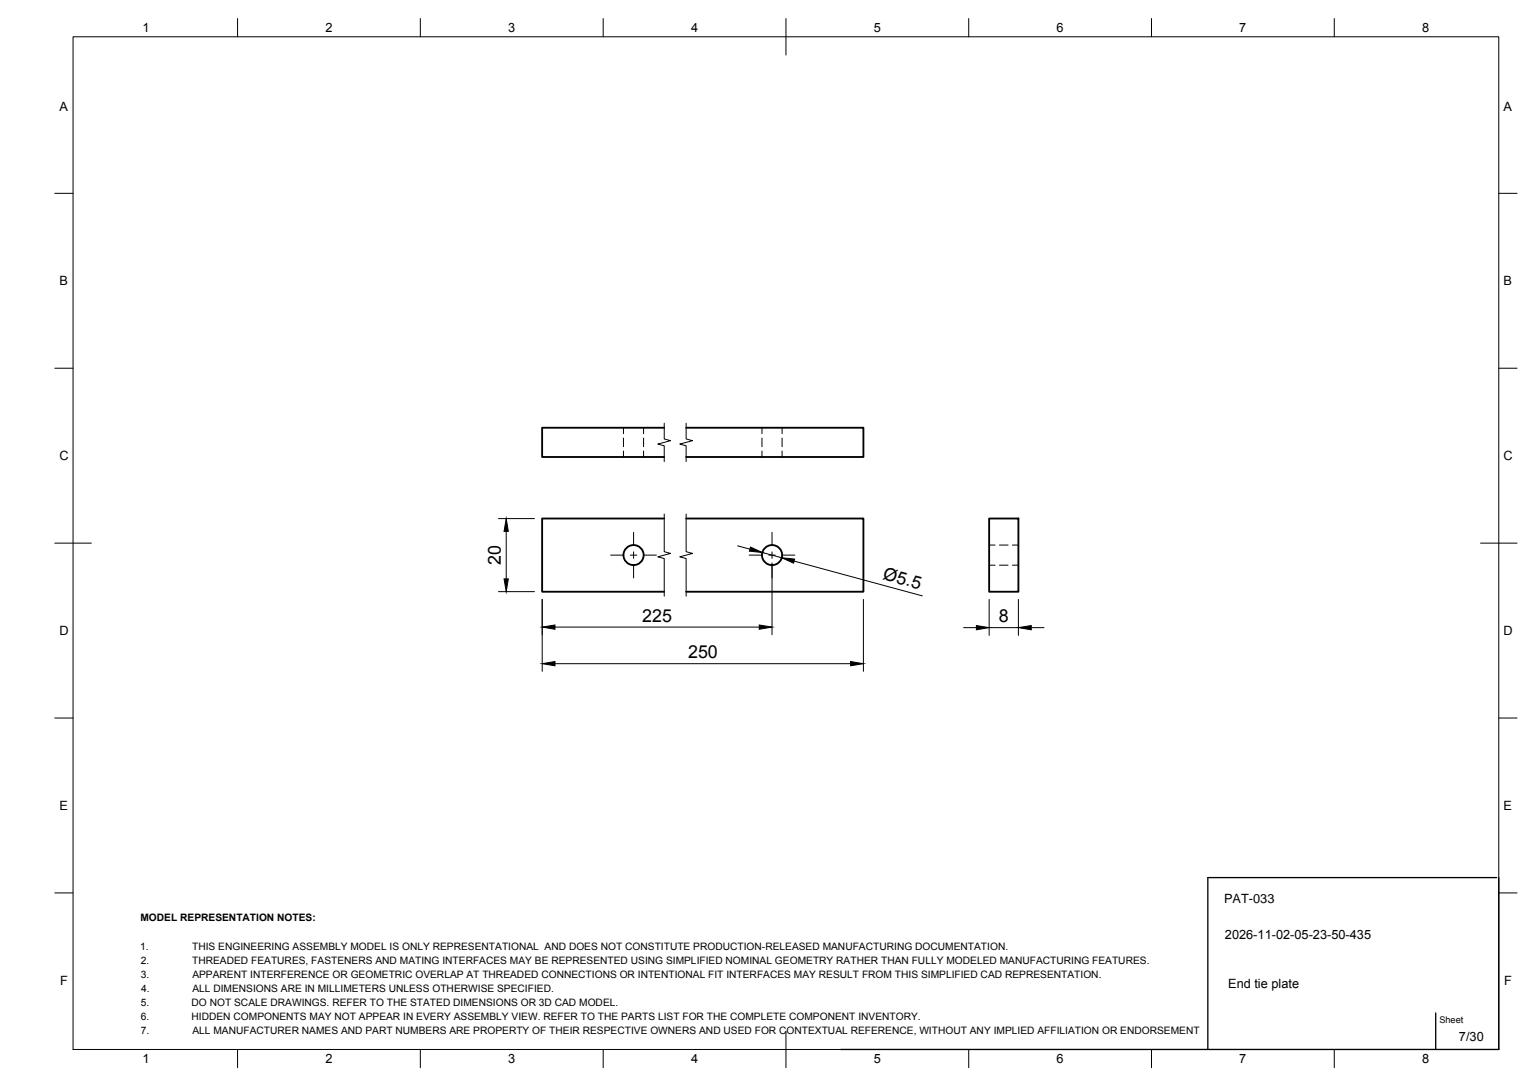
ISO-10303-21;
HEADER;
/* Generated by software containing ST-Developer
 * from STEP Tools, Inc. (www.steptools.com) 
 */

FILE_DESCRIPTION(
/* description */ ('Dual-rail gantry carriage'),
/* implementation_level */ '2;1');

FILE_NAME(
/* name */ 'End tie plate.step',
/* time_stamp */ '2026-10-27T10:49:15-07:00',
/* author */ (''),
/* organization */ (''),
/* preprocessor_version */ 'ST-DEVELOPER v20.2',
/* originating_system */ 'Autodesk Translation Framework v15.17.0.0',
/* authorisation */ '');

FILE_SCHEMA (('AUTOMOTIVE_DESIGN { 1 0 10303 214 3 1 1 }'));
ENDSEC;

DATA;
#10=MECHANICAL_DESIGN_GEOMETRIC_PRESENTATION_REPRESENTATION('',(#587),#12804);
#525=SHAPE_REPRESENTATION_RELATIONSHIP('SRR','None',#13003,#556);
#556=ADVANCED_BREP_SHAPE_REPRESENTATION('',(#618),#12773);
#587=STYLED_ITEM('',(#13233),#618);
#618=MANIFOLD_SOLID_BREP('Body1',#7365);
#666=FACE_BOUND('',#1492,.T.);
#667=FACE_BOUND('',#1493,.T.);
#668=FACE_BOUND('',#1495,.T.);
#669=FACE_BOUND('',#1496,.T.);
#776=PLANE('',#7800);
#777=PLANE('',#7801);
#778=PLANE('',#7802);
#779=PLANE('',#7803);
#780=PLANE('',#7804);
#781=PLANE('',#7805);
#1072=FACE_OUTER_BOUND('',#1485,.T.);
#1073=FACE_OUTER_BOUND('',#1486,.T.);
#1074=FACE_OUTER_BOUND('',#1487,.T.);
#1075=FACE_OUTER_BOUND('',#1488,.T.);
#1076=FACE_OUTER_BOUND('',#1489,.T.);
#1077=FACE_OUTER_BOUND('',#1490,.T.);
#1078=FACE_OUTER_BOUND('',#1491,.T.);
#1079=FACE_OUTER_BOUND('',#1494,.T.);
#1485=EDGE_LOOP('',(#5187,#5188,#5189,#5190));
#1486=EDGE_LOOP('',(#5191,#5192,#5193,#5194));
#1487=EDGE_LOOP('',(#5195,#5196,#5197,#5198));
#1488=EDGE_LOOP('',(#5199,#5200,#5201,#5202));
#1489=EDGE_LOOP('',(#5203,#5204,#5205,#5206));
#1490=EDGE_LOOP('',(#5207,#5208,#5209,#5210));
#1491=EDGE_LOOP('',(#5211,#5212,#5213,#5214));
#1492=EDGE_LOOP('',(#5215));
#1493=EDGE_LOOP('',(#5216));
#1494=EDGE_LOOP('',(#5217,#5218,#5219,#5220));
#1495=EDGE_LOOP('',(#5221));
#1496=EDGE_LOOP('',(#5222));
#1984=LINE('',#10821,#2693);
#1985=LINE('',#10827,#2694);
#1986=LINE('',#10832,#2695);
#1987=LINE('',#10834,#2696);
#1988=LINE('',#10836,#2697);
#1989=LINE('',#10837,#2698);
#1990=LINE('',#10840,#2699);
#1991=LINE('',#10842,#2700);
#1992=LINE('',#10843,#2701);
#1993=LINE('',#10846,#2702);
#1994=LINE('',#10848,#2703);
#1995=LINE('',#10849,#2704);
#1996=LINE('',#10851,#2705);
#1997=LINE('',#10852,#2706);
#2693=VECTOR('',#8633,0.275);
#2694=VECTOR('',#8640,0.275);
#2695=VECTOR('',#8645,1.);
#2696=VECTOR('',#8646,1.);
#2697=VECTOR('',#8647,1.);
#2698=VECTOR('',#8648,1.);
#2699=VECTOR('',#8651,1.);
#2700=VECTOR('',#8652,1.);
#2701=VECTOR('',#8653,1.);
#2702=VECTOR('',#8656,1.);
#2703=VECTOR('',#8657,1.);
#2704=VECTOR('',#8658,1.);
#2705=VECTOR('',#8661,1.);
#2706=VECTOR('',#8662,1.);
#3390=CIRCLE('',#7795,0.275);
#3391=CIRCLE('',#7796,0.275);
#3392=CIRCLE('',#7798,0.275);
#3393=CIRCLE('',#7799,0.275);
#3606=VERTEX_POINT('',#10818);
#3607=VERTEX_POINT('',#10820);
#3608=VERTEX_POINT('',#10824);
#3609=VERTEX_POINT('',#10826);
#3610=VERTEX_POINT('',#10830);
#3611=VERTEX_POINT('',#10831);
#3612=VERTEX_POINT('',#10833);
#3613=VERTEX_POINT('',#10835);
#3614=VERTEX_POINT('',#10839);
#3615=VERTEX_POINT('',#10841);
#3616=VERTEX_POINT('',#10845);
#3617=VERTEX_POINT('',#10847);
#4216=EDGE_CURVE('',#3606,#3606,#3390,.T.);
#4217=EDGE_CURVE('',#3606,#3607,#1984,.T.);
#4218=EDGE_CURVE('',#3607,#3607,#3391,.T.);
#4219=EDGE_CURVE('',#3608,#3608,#3392,.T.);
#4220=EDGE_CURVE('',#3608,#3609,#1985,.T.);
#4221=EDGE_CURVE('',#3609,#3609,#3393,.T.);
#4222=EDGE_CURVE('',#3610,#3611,#1986,.T.);
#4223=EDGE_CURVE('',#3611,#3612,#1987,.T.);
#4224=EDGE_CURVE('',#3613,#3612,#1988,.T.);
#4225=EDGE_CURVE('',#3610,#3613,#1989,.T.);
#4226=EDGE_CURVE('',#3614,#3610,#1990,.T.);
#4227=EDGE_CURVE('',#3615,#3613,#1991,.T.);
#4228=EDGE_CURVE('',#3614,#3615,#1992,.T.);
#4229=EDGE_CURVE('',#3616,#3614,#1993,.T.);
#4230=EDGE_CURVE('',#3617,#3615,#1994,.T.);
#4231=EDGE_CURVE('',#3616,#3617,#1995,.T.);
#4232=EDGE_CURVE('',#3611,#3616,#1996,.T.);
#4233=EDGE_CURVE('',#3612,#3617,#1997,.T.);
#5187=ORIENTED_EDGE('',*,*,#4216,.F.);
#5188=ORIENTED_EDGE('',*,*,#4217,.T.);
#5189=ORIENTED_EDGE('',*,*,#4218,.F.);
#5190=ORIENTED_EDGE('',*,*,#4217,.F.);
#5191=ORIENTED_EDGE('',*,*,#4219,.F.);
#5192=ORIENTED_EDGE('',*,*,#4220,.T.);
#5193=ORIENTED_EDGE('',*,*,#4221,.F.);
#5194=ORIENTED_EDGE('',*,*,#4220,.F.);
#5195=ORIENTED_EDGE('',*,*,#4222,.T.);
#5196=ORIENTED_EDGE('',*,*,#4223,.T.);
#5197=ORIENTED_EDGE('',*,*,#4224,.F.);
#5198=ORIENTED_EDGE('',*,*,#4225,.F.);
#5199=ORIENTED_EDGE('',*,*,#4226,.T.);
#5200=ORIENTED_EDGE('',*,*,#4225,.T.);
#5201=ORIENTED_EDGE('',*,*,#4227,.F.);
#5202=ORIENTED_EDGE('',*,*,#4228,.F.);
#5203=ORIENTED_EDGE('',*,*,#4229,.T.);
#5204=ORIENTED_EDGE('',*,*,#4228,.T.);
#5205=ORIENTED_EDGE('',*,*,#4230,.F.);
#5206=ORIENTED_EDGE('',*,*,#4231,.F.);
#5207=ORIENTED_EDGE('',*,*,#4232,.T.);
#5208=ORIENTED_EDGE('',*,*,#4231,.T.);
#5209=ORIENTED_EDGE('',*,*,#4233,.F.);
#5210=ORIENTED_EDGE('',*,*,#4223,.F.);
#5211=ORIENTED_EDGE('',*,*,#4233,.T.);
#5212=ORIENTED_EDGE('',*,*,#4230,.T.);
#5213=ORIENTED_EDGE('',*,*,#4227,.T.);
#5214=ORIENTED_EDGE('',*,*,#4224,.T.);
#5215=ORIENTED_EDGE('',*,*,#4218,.T.);
#5216=ORIENTED_EDGE('',*,*,#4221,.T.);
#5217=ORIENTED_EDGE('',*,*,#4232,.F.);
#5218=ORIENTED_EDGE('',*,*,#4222,.F.);
#5219=ORIENTED_EDGE('',*,*,#4226,.F.);
#5220=ORIENTED_EDGE('',*,*,#4229,.F.);
#5221=ORIENTED_EDGE('',*,*,#4216,.T.);
#5222=ORIENTED_EDGE('',*,*,#4219,.T.);
#6901=CYLINDRICAL_SURFACE('',#7794,0.275);
#6902=CYLINDRICAL_SURFACE('',#7797,0.275);
#6998=ADVANCED_FACE('',(#1072),#6901,.F.);
#6999=ADVANCED_FACE('',(#1073),#6902,.F.);
#7000=ADVANCED_FACE('',(#1074),#776,.T.);
#7001=ADVANCED_FACE('',(#1075),#777,.T.);
#7002=ADVANCED_FACE('',(#1076),#778,.T.);
#7003=ADVANCED_FACE('',(#1077),#779,.T.);
#7004=ADVANCED_FACE('',(#1078,#666,#667),#780,.T.);
#7005=ADVANCED_FACE('',(#1079,#668,#669),#781,.F.);
#7365=CLOSED_SHELL('',(#6998,#6999,#7000,#7001,#7002,#7003,#7004,#7005));
#7793=AXIS2_PLACEMENT_3D('',#10816,#8627,#8628);
#7794=AXIS2_PLACEMENT_3D('',#10817,#8629,#8630);
#7795=AXIS2_PLACEMENT_3D('',#10819,#8631,#8632);
#7796=AXIS2_PLACEMENT_3D('',#10822,#8634,#8635);
#7797=AXIS2_PLACEMENT_3D('',#10823,#8636,#8637);
#7798=AXIS2_PLACEMENT_3D('',#10825,#8638,#8639);
#7799=AXIS2_PLACEMENT_3D('',#10828,#8641,#8642);
#7800=AXIS2_PLACEMENT_3D('',#10829,#8643,#8644);
#7801=AXIS2_PLACEMENT_3D('',#10838,#8649,#8650);
#7802=AXIS2_PLACEMENT_3D('',#10844,#8654,#8655);
#7803=AXIS2_PLACEMENT_3D('',#10850,#8659,#8660);
#7804=AXIS2_PLACEMENT_3D('',#10853,#8663,#8664);
#7805=AXIS2_PLACEMENT_3D('',#10854,#8665,#8666);
#8627=DIRECTION('axis',(0.,0.,1.));
#8628=DIRECTION('refdir',(1.,0.,0.));
#8629=DIRECTION('center_axis',(0.,0.,1.));
#8630=DIRECTION('ref_axis',(1.,0.,0.));
#8631=DIRECTION('center_axis',(0.,0.,1.));
#8632=DIRECTION('ref_axis',(1.,0.,0.));
#8633=DIRECTION('',(0.,0.,1.));
#8634=DIRECTION('center_axis',(0.,0.,-1.));
#8635=DIRECTION('ref_axis',(1.,0.,0.));
#8636=DIRECTION('center_axis',(0.,0.,1.));
#8637=DIRECTION('ref_axis',(1.,0.,0.));
#8638=DIRECTION('center_axis',(0.,0.,1.));
#8639=DIRECTION('ref_axis',(1.,0.,0.));
#8640=DIRECTION('',(0.,0.,1.));
#8641=DIRECTION('center_axis',(0.,0.,-1.));
#8642=DIRECTION('ref_axis',(1.,0.,0.));
#8643=DIRECTION('center_axis',(0.,1.,0.));
#8644=DIRECTION('ref_axis',(-1.,0.,0.));
#8645=DIRECTION('',(-1.,0.,0.));
#8646=DIRECTION('',(0.,0.,1.));
#8647=DIRECTION('',(-1.,0.,0.));
#8648=DIRECTION('',(0.,0.,1.));
#8649=DIRECTION('center_axis',(1.,0.,0.));
#8650=DIRECTION('ref_axis',(0.,1.,0.));
#8651=DIRECTION('',(0.,1.,0.));
#8652=DIRECTION('',(0.,1.,0.));
#8653=DIRECTION('',(0.,0.,1.));
#8654=DIRECTION('center_axis',(0.,-1.,0.));
#8655=DIRECTION('ref_axis',(1.,0.,0.));
#8656=DIRECTION('',(1.,0.,0.));
#8657=DIRECTION('',(1.,0.,0.));
#8658=DIRECTION('',(0.,0.,1.));
#8659=DIRECTION('center_axis',(-1.,0.,0.));
#8660=DIRECTION('ref_axis',(0.,-1.,0.));
#8661=DIRECTION('',(0.,-1.,0.));
#8662=DIRECTION('',(0.,-1.,0.));
#8663=DIRECTION('center_axis',(0.,0.,1.));
#8664=DIRECTION('ref_axis',(1.,0.,0.));
#8665=DIRECTION('center_axis',(0.,0.,1.));
#8666=DIRECTION('ref_axis',(1.,0.,0.));
#10816=CARTESIAN_POINT('',(0.,0.,0.));
#10817=CARTESIAN_POINT('Origin',(1.,-10.,-0.9));
#10818=CARTESIAN_POINT('',(0.725,-10.,2.));
#10819=CARTESIAN_POINT('Origin',(1.,-10.,2.));
#10820=CARTESIAN_POINT('',(0.725,-10.,2.8));
#10821=CARTESIAN_POINT('',(0.725,-10.,-0.9));
#10822=CARTESIAN_POINT('Origin',(1.,-10.,2.8));
#10823=CARTESIAN_POINT('Origin',(1.,10.,-0.9));
#10824=CARTESIAN_POINT('',(0.725,10.,2.));
#10825=CARTESIAN_POINT('Origin',(1.,10.,2.));
#10826=CARTESIAN_POINT('',(0.725,10.,2.8));
#10827=CARTESIAN_POINT('',(0.725,10.,-0.9));
#10828=CARTESIAN_POINT('Origin',(1.,10.,2.8));
#10829=CARTESIAN_POINT('Origin',(2.,12.5,2.));
#10830=CARTESIAN_POINT('',(2.,12.5,2.));
#10831=CARTESIAN_POINT('',(0.,12.5,2.));
#10832=CARTESIAN_POINT('',(2.,12.5,2.));
#10833=CARTESIAN_POINT('',(0.,12.5,2.8));
#10834=CARTESIAN_POINT('',(0.,12.5,2.));
#10835=CARTESIAN_POINT('',(2.,12.5,2.8));
#10836=CARTESIAN_POINT('',(2.,12.5,2.8));
#10837=CARTESIAN_POINT('',(2.,12.5,2.));
#10838=CARTESIAN_POINT('Origin',(2.,-12.5,2.));
#10839=CARTESIAN_POINT('',(2.,-12.5,2.));
#10840=CARTESIAN_POINT('',(2.,-12.5,2.));
#10841=CARTESIAN_POINT('',(2.,-12.5,2.8));
#10842=CARTESIAN_POINT('',(2.,-12.5,2.8));
#10843=CARTESIAN_POINT('',(2.,-12.5,2.));
#10844=CARTESIAN_POINT('Origin',(0.,-12.5,2.));
#10845=CARTESIAN_POINT('',(0.,-12.5,2.));
#10846=CARTESIAN_POINT('',(0.,-12.5,2.));
#10847=CARTESIAN_POINT('',(0.,-12.5,2.8));
#10848=CARTESIAN_POINT('',(0.,-12.5,2.8));
#10849=CARTESIAN_POINT('',(0.,-12.5,2.));
#10850=CARTESIAN_POINT('Origin',(0.,12.5,2.));
#10851=CARTESIAN_POINT('',(0.,12.5,2.));
#10852=CARTESIAN_POINT('',(0.,12.5,2.8));
#10853=CARTESIAN_POINT('Origin',(1.,0.,2.8));
#10854=CARTESIAN_POINT('Origin',(1.,0.,2.));
#12737=UNCERTAINTY_MEASURE_WITH_UNIT(LENGTH_MEASURE(0.001),#12805,
'DISTANCE_ACCURACY_VALUE',
'Maximum model space distance between geometric entities at asserted c
onnectivities');
#12768=UNCERTAINTY_MEASURE_WITH_UNIT(LENGTH_MEASURE(0.001),#12805,
'DISTANCE_ACCURACY_VALUE',
'Maximum model space distance between geometric entities at asserted c
onnectivities');
#12773=(
GEOMETRIC_REPRESENTATION_CONTEXT(3)
GLOBAL_UNCERTAINTY_ASSIGNED_CONTEXT((#12737))
GLOBAL_UNIT_ASSIGNED_CONTEXT((#12805,#12807,#12808))
REPRESENTATION_CONTEXT('','3D')
);
#12804=(
GEOMETRIC_REPRESENTATION_CONTEXT(3)
GLOBAL_UNCERTAINTY_ASSIGNED_CONTEXT((#12768))
GLOBAL_UNIT_ASSIGNED_CONTEXT((#12805,#12807,#12808))
REPRESENTATION_CONTEXT('','3D')
);
#12805=(
LENGTH_UNIT()
NAMED_UNIT(*)
SI_UNIT(.CENTI.,.METRE.)
);
#12807=(
NAMED_UNIT(*)
PLANE_ANGLE_UNIT()
SI_UNIT($,.RADIAN.)
);
#12808=(
NAMED_UNIT(*)
SI_UNIT($,.STERADIAN.)
SOLID_ANGLE_UNIT()
);
#12813=SHAPE_DEFINITION_REPRESENTATION(#12848,#13003);
#12848=PRODUCT_DEFINITION_SHAPE('',$,#13039);
#13003=SHAPE_REPRESENTATION('',(#7793),#12773);
#13034=PRODUCT_DEFINITION_CONTEXT('part definition',#13141,'design');
#13039=PRODUCT_DEFINITION('End tie plate','End tie plate',#13074,#13034);
#13074=PRODUCT_DEFINITION_FORMATION('',$,#13147);
#13141=APPLICATION_CONTEXT(
'Core Data for Automotive Mechanical Design Process');
#13142=PRODUCT_CONTEXT('part definition',#13141,'mechanical');
#13147=PRODUCT('End tie plate','End tie plate','End tie plate',(#13142));
#13227=COLOUR_RGB('Light Blue',0.38,0.62,0.78);
#13228=FILL_AREA_STYLE_COLOUR('',#13227);
#13229=FILL_AREA_STYLE('',(#13228));
#13230=SURFACE_STYLE_FILL_AREA(#13229);
#13231=SURFACE_SIDE_STYLE('',(#13230));
#13232=SURFACE_STYLE_USAGE(.BOTH.,#13231);
#13233=PRESENTATION_STYLE_ASSIGNMENT((#13232));
ENDSEC;
END-ISO-10303-21;
